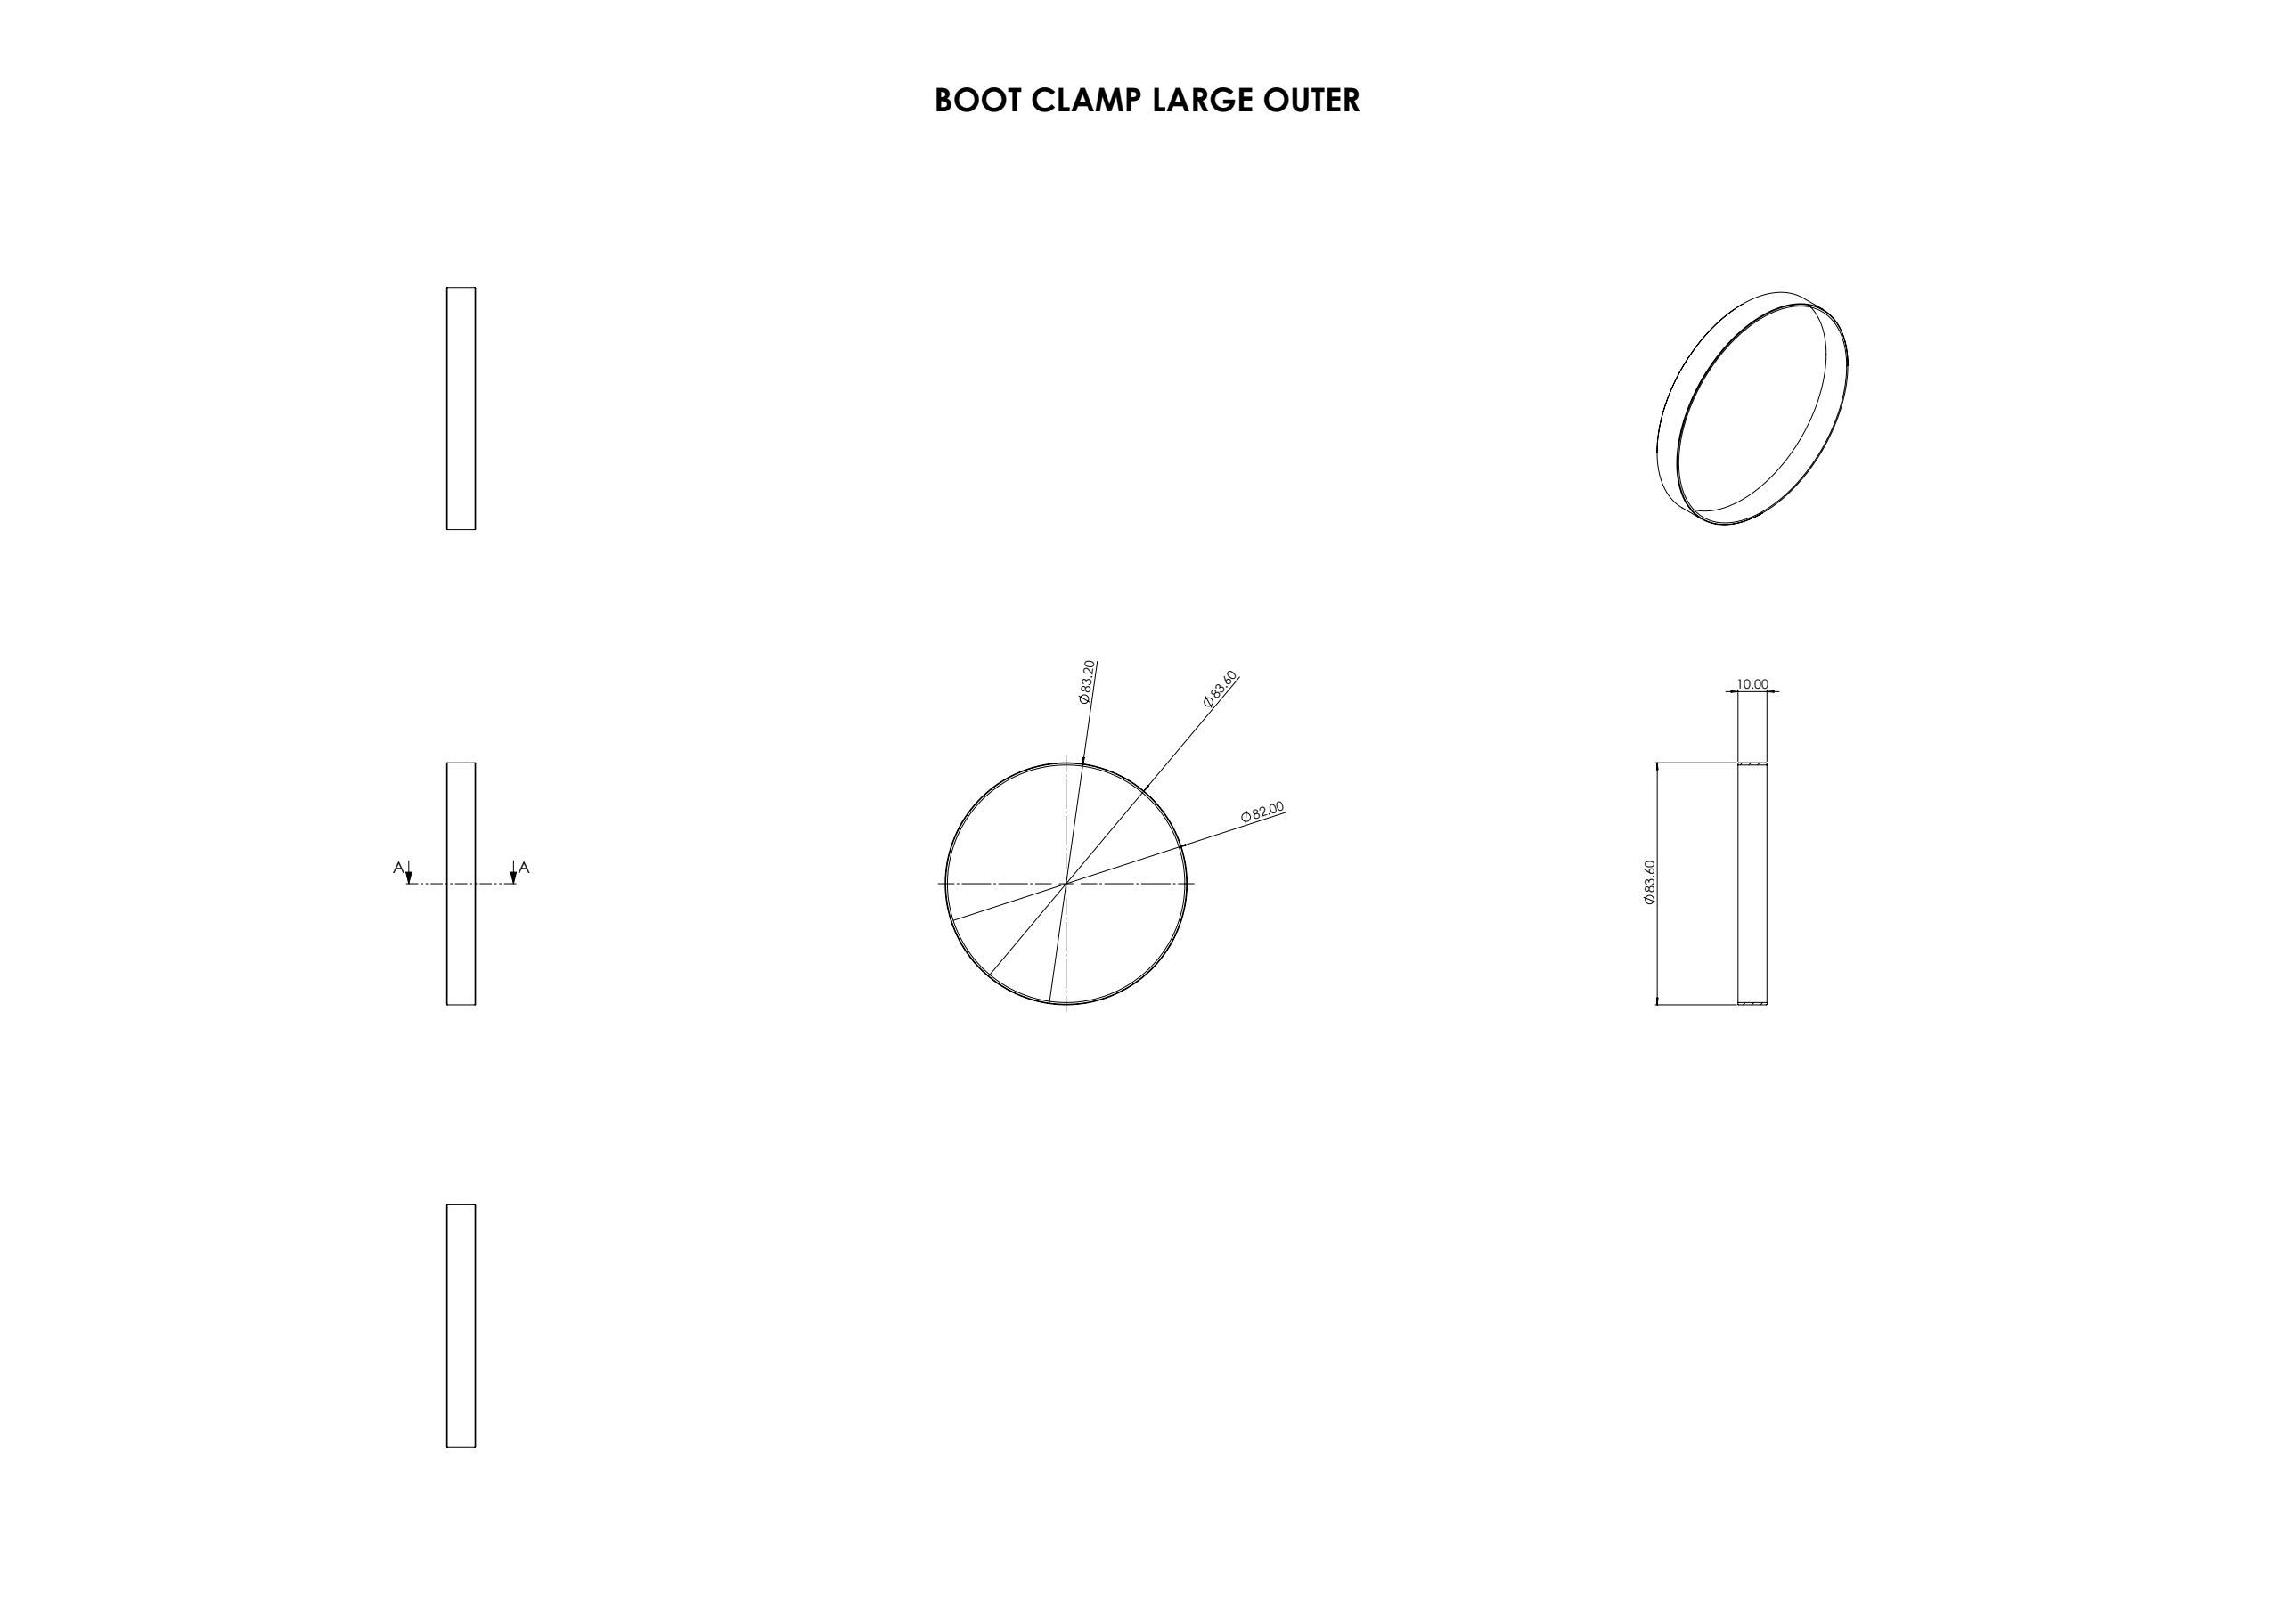
ISO-10303-21;
HEADER;
/* Generated by software containing ST-Developer
 * from STEP Tools, Inc. (www.steptools.com) 
 */

FILE_DESCRIPTION(
/* description */ (''),
/* implementation_level */ '2;1');

FILE_NAME(
/* name */ '08_Boot_Clamp_Large_Outer.step',
/* time_stamp */ '2026-10-11T12:57:03-07:00',
/* author */ (''),
/* organization */ (''),
/* preprocessor_version */ 'ST-DEVELOPER v20.2',
/* originating_system */ 'Autodesk Translation Framework v15.15.0.0',
/* authorisation */ '');

FILE_SCHEMA (('AUTOMOTIVE_DESIGN { 1 0 10303 214 3 1 1 }'));
ENDSEC;

DATA;
#10=MECHANICAL_DESIGN_GEOMETRIC_PRESENTATION_REPRESENTATION('',(#263),#90374);
#229=SHAPE_REPRESENTATION_RELATIONSHIP('SRR','None',#90448,#246);
#246=ADVANCED_BREP_SHAPE_REPRESENTATION('',(#280),#90364);
#263=STYLED_ITEM('',(#90673),#280);
#280=MANIFOLD_SOLID_BREP('Body1',#40352);
#689=CONICAL_SURFACE('',#43820,41.7,0.785398163397515);
#690=CONICAL_SURFACE('',#43825,41.7,0.785398163397559);
#1069=FACE_BOUND('',#6247,.T.);
#1070=FACE_BOUND('',#6250,.T.);
#1439=PLANE('',#43827);
#1440=PLANE('',#43831);
#3817=FACE_OUTER_BOUND('',#6243,.T.);
#3818=FACE_OUTER_BOUND('',#6244,.T.);
#3819=FACE_OUTER_BOUND('',#6245,.T.);
#3820=FACE_OUTER_BOUND('',#6246,.T.);
#3821=FACE_OUTER_BOUND('',#6248,.T.);
#3822=FACE_OUTER_BOUND('',#6249,.T.);
#6243=EDGE_LOOP('',(#33311,#33312,#33313,#33314));
#6244=EDGE_LOOP('',(#33315,#33316,#33317,#33318));
#6245=EDGE_LOOP('',(#33319,#33320,#33321,#33322));
#6246=EDGE_LOOP('',(#33323));
#6247=EDGE_LOOP('',(#33324));
#6248=EDGE_LOOP('',(#33325,#33326,#33327,#33328));
#6249=EDGE_LOOP('',(#33329));
#6250=EDGE_LOOP('',(#33330));
#8693=CIRCLE('',#43821,41.8);
#8694=CIRCLE('',#43822,41.6);
#8695=CIRCLE('',#43824,41.8);
#8696=CIRCLE('',#43826,41.6);
#8697=CIRCLE('',#43828,41.);
#8698=CIRCLE('',#43830,41.);
#11847=LINE('',#82980,#14341);
#11848=LINE('',#82985,#14342);
#11849=LINE('',#82989,#14343);
#11850=LINE('',#82995,#14344);
#14341=VECTOR('',#53329,41.7);
#14342=VECTOR('',#53336,41.8);
#14343=VECTOR('',#53341,41.7);
#14344=VECTOR('',#53348,41.);
#17788=VERTEX_POINT('',#82977);
#17789=VERTEX_POINT('',#82979);
#17790=VERTEX_POINT('',#82983);
#17791=VERTEX_POINT('',#82987);
#17792=VERTEX_POINT('',#82991);
#17793=VERTEX_POINT('',#82994);
#23167=EDGE_CURVE('',#17788,#17788,#8693,.T.);
#23168=EDGE_CURVE('',#17788,#17789,#11847,.T.);
#23169=EDGE_CURVE('',#17789,#17789,#8694,.T.);
#23170=EDGE_CURVE('',#17790,#17790,#8695,.T.);
#23171=EDGE_CURVE('',#17790,#17788,#11848,.T.);
#23172=EDGE_CURVE('',#17791,#17791,#8696,.T.);
#23173=EDGE_CURVE('',#17791,#17790,#11849,.T.);
#23174=EDGE_CURVE('',#17792,#17792,#8697,.T.);
#23175=EDGE_CURVE('',#17792,#17793,#11850,.T.);
#23176=EDGE_CURVE('',#17793,#17793,#8698,.T.);
#33311=ORIENTED_EDGE('',*,*,#23167,.F.);
#33312=ORIENTED_EDGE('',*,*,#23168,.T.);
#33313=ORIENTED_EDGE('',*,*,#23169,.T.);
#33314=ORIENTED_EDGE('',*,*,#23168,.F.);
#33315=ORIENTED_EDGE('',*,*,#23170,.F.);
#33316=ORIENTED_EDGE('',*,*,#23171,.T.);
#33317=ORIENTED_EDGE('',*,*,#23167,.T.);
#33318=ORIENTED_EDGE('',*,*,#23171,.F.);
#33319=ORIENTED_EDGE('',*,*,#23172,.F.);
#33320=ORIENTED_EDGE('',*,*,#23173,.T.);
#33321=ORIENTED_EDGE('',*,*,#23170,.T.);
#33322=ORIENTED_EDGE('',*,*,#23173,.F.);
#33323=ORIENTED_EDGE('',*,*,#23172,.T.);
#33324=ORIENTED_EDGE('',*,*,#23174,.F.);
#33325=ORIENTED_EDGE('',*,*,#23174,.T.);
#33326=ORIENTED_EDGE('',*,*,#23175,.T.);
#33327=ORIENTED_EDGE('',*,*,#23176,.F.);
#33328=ORIENTED_EDGE('',*,*,#23175,.F.);
#33329=ORIENTED_EDGE('',*,*,#23169,.F.);
#33330=ORIENTED_EDGE('',*,*,#23176,.T.);
#37774=CYLINDRICAL_SURFACE('',#43823,41.8);
#37775=CYLINDRICAL_SURFACE('',#43829,41.);
#39620=ADVANCED_FACE('',(#3817),#689,.T.);
#39621=ADVANCED_FACE('',(#3818),#37774,.T.);
#39622=ADVANCED_FACE('',(#3819),#690,.T.);
#39623=ADVANCED_FACE('',(#3820,#1069),#1439,.T.);
#39624=ADVANCED_FACE('',(#3821),#37775,.F.);
#39625=ADVANCED_FACE('',(#3822,#1070),#1440,.T.);
#40352=CLOSED_SHELL('',(#39620,#39621,#39622,#39623,#39624,#39625));
#43819=AXIS2_PLACEMENT_3D('',#82975,#53323,#53324);
#43820=AXIS2_PLACEMENT_3D('',#82976,#53325,#53326);
#43821=AXIS2_PLACEMENT_3D('',#82978,#53327,#53328);
#43822=AXIS2_PLACEMENT_3D('',#82981,#53330,#53331);
#43823=AXIS2_PLACEMENT_3D('',#82982,#53332,#53333);
#43824=AXIS2_PLACEMENT_3D('',#82984,#53334,#53335);
#43825=AXIS2_PLACEMENT_3D('',#82986,#53337,#53338);
#43826=AXIS2_PLACEMENT_3D('',#82988,#53339,#53340);
#43827=AXIS2_PLACEMENT_3D('',#82990,#53342,#53343);
#43828=AXIS2_PLACEMENT_3D('',#82992,#53344,#53345);
#43829=AXIS2_PLACEMENT_3D('',#82993,#53346,#53347);
#43830=AXIS2_PLACEMENT_3D('',#82996,#53349,#53350);
#43831=AXIS2_PLACEMENT_3D('',#82997,#53351,#53352);
#53323=DIRECTION('axis',(0.,0.,1.));
#53324=DIRECTION('refdir',(1.,0.,0.));
#53325=DIRECTION('center_axis',(1.,0.,0.));
#53326=DIRECTION('ref_axis',(0.,1.,0.));
#53327=DIRECTION('center_axis',(1.,0.,0.));
#53328=DIRECTION('ref_axis',(0.,0.,-1.));
#53329=DIRECTION('',(-0.7071067811865,0.707106781186595,8.65956056235551E-17));
#53330=DIRECTION('center_axis',(1.,0.,0.));
#53331=DIRECTION('ref_axis',(0.,0.,-1.));
#53332=DIRECTION('center_axis',(1.,0.,0.));
#53333=DIRECTION('ref_axis',(0.,1.,0.));
#53334=DIRECTION('center_axis',(1.,0.,0.));
#53335=DIRECTION('ref_axis',(0.,0.,-1.));
#53336=DIRECTION('',(-1.,0.,0.));
#53337=DIRECTION('center_axis',(-1.,0.,0.));
#53338=DIRECTION('ref_axis',(0.,1.,0.));
#53339=DIRECTION('center_axis',(1.,0.,0.));
#53340=DIRECTION('ref_axis',(0.,0.,-1.));
#53341=DIRECTION('',(-0.707106781186469,-0.707106781186626,-8.6595605623559E-17));
#53342=DIRECTION('center_axis',(1.,0.,0.));
#53343=DIRECTION('ref_axis',(0.,0.,-1.));
#53344=DIRECTION('center_axis',(1.,0.,0.));
#53345=DIRECTION('ref_axis',(0.,0.,-1.));
#53346=DIRECTION('center_axis',(1.,0.,0.));
#53347=DIRECTION('ref_axis',(0.,1.,0.));
#53348=DIRECTION('',(-1.,0.,0.));
#53349=DIRECTION('center_axis',(1.,0.,0.));
#53350=DIRECTION('ref_axis',(0.,0.,-1.));
#53351=DIRECTION('center_axis',(-1.,0.,0.));
#53352=DIRECTION('ref_axis',(0.,0.,1.));
#82975=CARTESIAN_POINT('',(0.,0.,0.));
#82976=CARTESIAN_POINT('Origin',(154.1,0.,0.));
#82977=CARTESIAN_POINT('',(154.2,-41.8,-5.11902362043594E-15));
#82978=CARTESIAN_POINT('Origin',(154.2,0.,0.));
#82979=CARTESIAN_POINT('',(154.,-41.6,-5.09453068445299E-15));
#82980=CARTESIAN_POINT('',(154.1,-41.7,-5.10677715244446E-15));
#82981=CARTESIAN_POINT('Origin',(154.,0.,0.));
#82982=CARTESIAN_POINT('Origin',(159.,0.,0.));
#82983=CARTESIAN_POINT('',(163.8,-41.8,-5.11902362043594E-15));
#82984=CARTESIAN_POINT('Origin',(163.8,0.,0.));
#82985=CARTESIAN_POINT('',(159.,-41.8,-5.11902362043594E-15));
#82986=CARTESIAN_POINT('Origin',(163.9,0.,0.));
#82987=CARTESIAN_POINT('',(164.,-41.6,-5.09453068445299E-15));
#82988=CARTESIAN_POINT('Origin',(164.,0.,0.));
#82989=CARTESIAN_POINT('',(163.9,-41.7,-5.10677715244446E-15));
#82990=CARTESIAN_POINT('Origin',(164.,41.,0.));
#82991=CARTESIAN_POINT('',(164.,-41.,-5.02105187650415E-15));
#82992=CARTESIAN_POINT('Origin',(164.,0.,0.));
#82993=CARTESIAN_POINT('Origin',(159.,0.,0.));
#82994=CARTESIAN_POINT('',(154.,-41.,-5.02105187650415E-15));
#82995=CARTESIAN_POINT('',(159.,-41.,-5.02105187650415E-15));
#82996=CARTESIAN_POINT('Origin',(154.,0.,0.));
#82997=CARTESIAN_POINT('Origin',(154.,41.6,0.));
#90345=UNCERTAINTY_MEASURE_WITH_UNIT(LENGTH_MEASURE(0.01),#90375,
'DISTANCE_ACCURACY_VALUE',
'Maximum model space distance between geometric entities at asserted c
onnectivities');
#90355=UNCERTAINTY_MEASURE_WITH_UNIT(LENGTH_MEASURE(0.01),#90375,
'DISTANCE_ACCURACY_VALUE',
'Maximum model space distance between geometric entities at asserted c
onnectivities');
#90364=(
GEOMETRIC_REPRESENTATION_CONTEXT(3)
GLOBAL_UNCERTAINTY_ASSIGNED_CONTEXT((#90345))
GLOBAL_UNIT_ASSIGNED_CONTEXT((#90375,#90377,#90378))
REPRESENTATION_CONTEXT('','3D')
);
#90374=(
GEOMETRIC_REPRESENTATION_CONTEXT(3)
GLOBAL_UNCERTAINTY_ASSIGNED_CONTEXT((#90355))
GLOBAL_UNIT_ASSIGNED_CONTEXT((#90375,#90377,#90378))
REPRESENTATION_CONTEXT('','3D')
);
#90375=(
LENGTH_UNIT()
NAMED_UNIT(*)
SI_UNIT(.MILLI.,.METRE.)
);
#90377=(
NAMED_UNIT(*)
PLANE_ANGLE_UNIT()
SI_UNIT($,.RADIAN.)
);
#90378=(
NAMED_UNIT(*)
SI_UNIT($,.STERADIAN.)
SOLID_ANGLE_UNIT()
);
#90387=SHAPE_DEFINITION_REPRESENTATION(#90405,#90448);
#90405=PRODUCT_DEFINITION_SHAPE('',$,#90467);
#90448=SHAPE_REPRESENTATION('',(#43819),#90364);
#90458=PRODUCT_DEFINITION_CONTEXT('part definition',#90514,'design');
#90467=PRODUCT_DEFINITION('2026-10-11-12-53-11-026',
'08_Boot_Clamp_Large_Outer',#90485,#90458);
#90485=PRODUCT_DEFINITION_FORMATION('',$,#90524);
#90514=APPLICATION_CONTEXT(
'Core Data for Automotive Mechanical Design Process');
#90515=PRODUCT_CONTEXT('part definition',#90514,'mechanical');
#90524=PRODUCT('2026-10-11-12-53-11-026','08_Boot_Clamp_Large_Outer',$,
(#90515));
#90667=COLOUR_RGB('Light Blue',0.38,0.62,0.78);
#90668=FILL_AREA_STYLE_COLOUR('',#90667);
#90669=FILL_AREA_STYLE('',(#90668));
#90670=SURFACE_STYLE_FILL_AREA(#90669);
#90671=SURFACE_SIDE_STYLE('',(#90670));
#90672=SURFACE_STYLE_USAGE(.BOTH.,#90671);
#90673=PRESENTATION_STYLE_ASSIGNMENT((#90672));
ENDSEC;
END-ISO-10303-21;
